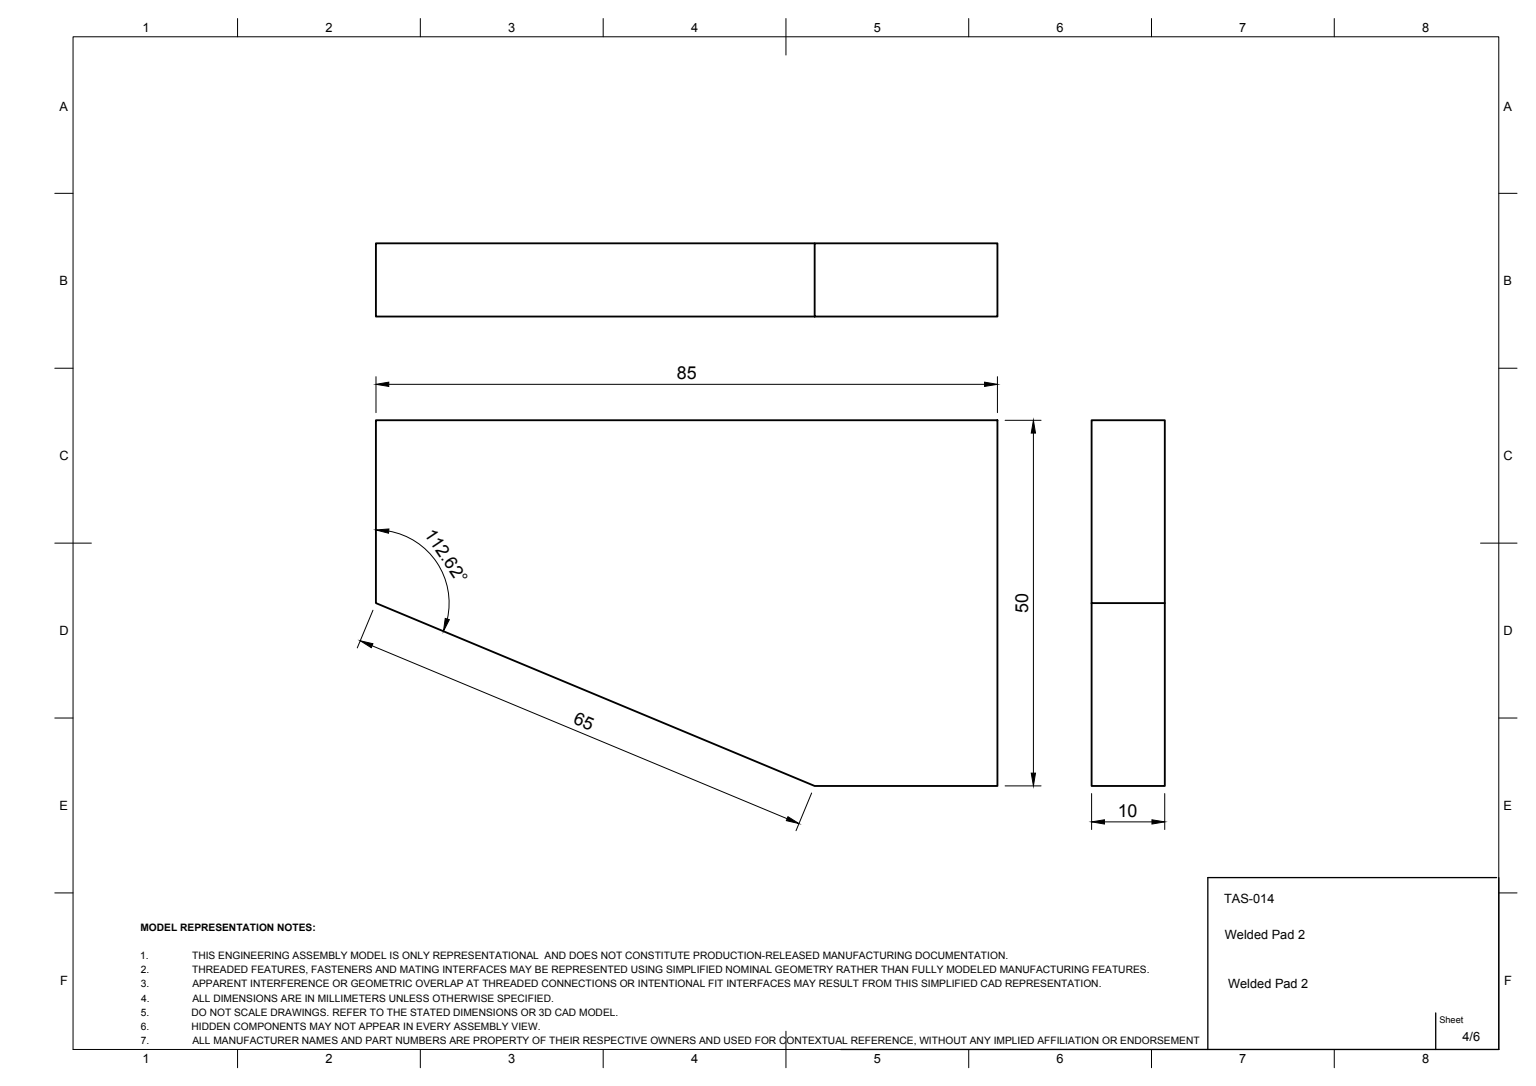
ISO-10303-21;
HEADER;
/* Generated by software containing ST-Developer
 * from STEP Tools, Inc. (www.steptools.com) 
 */

FILE_DESCRIPTION(
/* description */ ('STEP AP214'),
/* implementation_level */ '2;1');

FILE_NAME(
/* name */ 'Welded Pad 2.step',
/* time_stamp */ '2026-11-15T15:22:30-08:00',
/* author */ (''),
/* organization */ (''),
/* preprocessor_version */ 'ST-DEVELOPER v20.2',
/* originating_system */ 'Autodesk Translation Framework v15.17.0.0',
/* authorisation */ '');

FILE_SCHEMA (('AUTOMOTIVE_DESIGN { 1 0 10303 214 3 1 1 }'));
ENDSEC;

DATA;
#10=MECHANICAL_DESIGN_GEOMETRIC_PRESENTATION_REPRESENTATION('',(#87),#3119);
#70=SHAPE_REPRESENTATION_RELATIONSHIP('SRR','None',#3152,#74);
#74=ADVANCED_BREP_SHAPE_REPRESENTATION('',(#94),#3118);
#87=STYLED_ITEM('',(#3178),#94);
#94=MANIFOLD_SOLID_BREP('Body1',#1806);
#293=FACE_OUTER_BOUND('',#394,.T.);
#294=FACE_OUTER_BOUND('',#395,.T.);
#295=FACE_OUTER_BOUND('',#396,.T.);
#296=FACE_OUTER_BOUND('',#397,.T.);
#297=FACE_OUTER_BOUND('',#398,.T.);
#298=FACE_OUTER_BOUND('',#399,.T.);
#299=FACE_OUTER_BOUND('',#400,.T.);
#394=EDGE_LOOP('',(#1616,#1617,#1618,#1619));
#395=EDGE_LOOP('',(#1620,#1621,#1622,#1623));
#396=EDGE_LOOP('',(#1624,#1625,#1626,#1627));
#397=EDGE_LOOP('',(#1628,#1629,#1630,#1631));
#398=EDGE_LOOP('',(#1632,#1633,#1634,#1635));
#399=EDGE_LOOP('',(#1636,#1637,#1638,#1639,#1640));
#400=EDGE_LOOP('',(#1641,#1642,#1643,#1644,#1645));
#561=LINE('',#3065,#736);
#562=LINE('',#3067,#737);
#563=LINE('',#3069,#738);
#564=LINE('',#3070,#739);
#565=LINE('',#3073,#740);
#566=LINE('',#3075,#741);
#567=LINE('',#3076,#742);
#568=LINE('',#3079,#743);
#569=LINE('',#3081,#744);
#570=LINE('',#3082,#745);
#571=LINE('',#3085,#746);
#572=LINE('',#3087,#747);
#573=LINE('',#3088,#748);
#574=LINE('',#3090,#749);
#575=LINE('',#3091,#750);
#736=VECTOR('',#2524,1000.);
#737=VECTOR('',#2525,1000.);
#738=VECTOR('',#2526,1000.);
#739=VECTOR('',#2527,1000.);
#740=VECTOR('',#2530,1000.);
#741=VECTOR('',#2531,1000.);
#742=VECTOR('',#2532,1000.);
#743=VECTOR('',#2535,1000.);
#744=VECTOR('',#2536,1000.);
#745=VECTOR('',#2537,1000.);
#746=VECTOR('',#2540,1000.);
#747=VECTOR('',#2541,1000.);
#748=VECTOR('',#2542,1000.);
#749=VECTOR('',#2545,1000.);
#750=VECTOR('',#2546,1000.);
#911=VERTEX_POINT('',#3063);
#912=VERTEX_POINT('',#3064);
#913=VERTEX_POINT('',#3066);
#914=VERTEX_POINT('',#3068);
#915=VERTEX_POINT('',#3072);
#916=VERTEX_POINT('',#3074);
#917=VERTEX_POINT('',#3078);
#918=VERTEX_POINT('',#3080);
#919=VERTEX_POINT('',#3084);
#920=VERTEX_POINT('',#3086);
#1153=EDGE_CURVE('',#911,#912,#561,.T.);
#1154=EDGE_CURVE('',#913,#912,#562,.T.);
#1155=EDGE_CURVE('',#914,#913,#563,.T.);
#1156=EDGE_CURVE('',#914,#911,#564,.T.);
#1157=EDGE_CURVE('',#912,#915,#565,.T.);
#1158=EDGE_CURVE('',#916,#915,#566,.T.);
#1159=EDGE_CURVE('',#913,#916,#567,.T.);
#1160=EDGE_CURVE('',#915,#917,#568,.T.);
#1161=EDGE_CURVE('',#918,#917,#569,.T.);
#1162=EDGE_CURVE('',#916,#918,#570,.T.);
#1163=EDGE_CURVE('',#917,#919,#571,.T.);
#1164=EDGE_CURVE('',#920,#919,#572,.T.);
#1165=EDGE_CURVE('',#918,#920,#573,.T.);
#1166=EDGE_CURVE('',#919,#911,#574,.T.);
#1167=EDGE_CURVE('',#920,#914,#575,.T.);
#1616=ORIENTED_EDGE('',*,*,#1153,.T.);
#1617=ORIENTED_EDGE('',*,*,#1154,.F.);
#1618=ORIENTED_EDGE('',*,*,#1155,.F.);
#1619=ORIENTED_EDGE('',*,*,#1156,.T.);
#1620=ORIENTED_EDGE('',*,*,#1157,.T.);
#1621=ORIENTED_EDGE('',*,*,#1158,.F.);
#1622=ORIENTED_EDGE('',*,*,#1159,.F.);
#1623=ORIENTED_EDGE('',*,*,#1154,.T.);
#1624=ORIENTED_EDGE('',*,*,#1160,.T.);
#1625=ORIENTED_EDGE('',*,*,#1161,.F.);
#1626=ORIENTED_EDGE('',*,*,#1162,.F.);
#1627=ORIENTED_EDGE('',*,*,#1158,.T.);
#1628=ORIENTED_EDGE('',*,*,#1163,.T.);
#1629=ORIENTED_EDGE('',*,*,#1164,.F.);
#1630=ORIENTED_EDGE('',*,*,#1165,.F.);
#1631=ORIENTED_EDGE('',*,*,#1161,.T.);
#1632=ORIENTED_EDGE('',*,*,#1166,.T.);
#1633=ORIENTED_EDGE('',*,*,#1156,.F.);
#1634=ORIENTED_EDGE('',*,*,#1167,.F.);
#1635=ORIENTED_EDGE('',*,*,#1164,.T.);
#1636=ORIENTED_EDGE('',*,*,#1155,.T.);
#1637=ORIENTED_EDGE('',*,*,#1159,.T.);
#1638=ORIENTED_EDGE('',*,*,#1162,.T.);
#1639=ORIENTED_EDGE('',*,*,#1165,.T.);
#1640=ORIENTED_EDGE('',*,*,#1167,.T.);
#1641=ORIENTED_EDGE('',*,*,#1153,.F.);
#1642=ORIENTED_EDGE('',*,*,#1166,.F.);
#1643=ORIENTED_EDGE('',*,*,#1163,.F.);
#1644=ORIENTED_EDGE('',*,*,#1160,.F.);
#1645=ORIENTED_EDGE('',*,*,#1157,.F.);
#1700=PLANE('',#2015);
#1701=PLANE('',#2016);
#1702=PLANE('',#2017);
#1703=PLANE('',#2018);
#1704=PLANE('',#2019);
#1705=PLANE('',#2020);
#1706=PLANE('',#2021);
#1793=ADVANCED_FACE('',(#293),#1700,.F.);
#1794=ADVANCED_FACE('',(#294),#1701,.F.);
#1795=ADVANCED_FACE('',(#295),#1702,.F.);
#1796=ADVANCED_FACE('',(#296),#1703,.F.);
#1797=ADVANCED_FACE('',(#297),#1704,.F.);
#1798=ADVANCED_FACE('',(#298),#1705,.F.);
#1799=ADVANCED_FACE('',(#299),#1706,.T.);
#1806=CLOSED_SHELL('',(#1793,#1794,#1795,#1796,#1797,#1798,#1799));
#2014=AXIS2_PLACEMENT_3D('',#3061,#2520,#2521);
#2015=AXIS2_PLACEMENT_3D('',#3062,#2522,#2523);
#2016=AXIS2_PLACEMENT_3D('',#3071,#2528,#2529);
#2017=AXIS2_PLACEMENT_3D('',#3077,#2533,#2534);
#2018=AXIS2_PLACEMENT_3D('',#3083,#2538,#2539);
#2019=AXIS2_PLACEMENT_3D('',#3089,#2543,#2544);
#2020=AXIS2_PLACEMENT_3D('',#3092,#2547,#2548);
#2021=AXIS2_PLACEMENT_3D('',#3093,#2549,#2550);
#2520=DIRECTION('axis',(0.,0.,1.));
#2521=DIRECTION('refdir',(1.,0.,0.));
#2522=DIRECTION('center_axis',(0.,1.,0.));
#2523=DIRECTION('ref_axis',(0.,0.,1.));
#2524=DIRECTION('',(1.,0.,0.));
#2525=DIRECTION('',(0.,0.,-1.));
#2526=DIRECTION('',(1.,0.,0.));
#2527=DIRECTION('',(0.,0.,-1.));
#2528=DIRECTION('center_axis',(-1.,2.77555756156289E-16,0.));
#2529=DIRECTION('ref_axis',(-2.77555756156289E-16,-1.,0.));
#2530=DIRECTION('',(2.77555756156289E-16,1.,0.));
#2531=DIRECTION('',(0.,0.,-1.));
#2532=DIRECTION('',(2.77555756156289E-16,1.,0.));
#2533=DIRECTION('center_axis',(-0.923076923076923,-0.384615384615385,0.));
#2534=DIRECTION('ref_axis',(0.384615384615385,-0.923076923076923,0.));
#2535=DIRECTION('',(-0.384615384615385,0.923076923076923,0.));
#2536=DIRECTION('',(0.,0.,-1.));
#2537=DIRECTION('',(-0.384615384615385,0.923076923076923,0.));
#2538=DIRECTION('center_axis',(0.,-1.,0.));
#2539=DIRECTION('ref_axis',(0.,0.,-1.));
#2540=DIRECTION('',(-1.,0.,0.));
#2541=DIRECTION('',(0.,0.,-1.));
#2542=DIRECTION('',(-1.,0.,0.));
#2543=DIRECTION('center_axis',(1.,0.,0.));
#2544=DIRECTION('ref_axis',(0.,0.,-1.));
#2545=DIRECTION('',(0.,-1.,0.));
#2546=DIRECTION('',(0.,-1.,0.));
#2547=DIRECTION('center_axis',(0.,0.,-1.));
#2548=DIRECTION('ref_axis',(-1.,0.,0.));
#2549=DIRECTION('center_axis',(0.,0.,-1.));
#2550=DIRECTION('ref_axis',(-1.,0.,0.));
#3061=CARTESIAN_POINT('',(0.,0.,0.));
#3062=CARTESIAN_POINT('Origin',(50.,0.,5.));
#3063=CARTESIAN_POINT('',(0.,0.,-5.));
#3064=CARTESIAN_POINT('',(50.,0.,-5.));
#3065=CARTESIAN_POINT('',(50.,0.,-5.));
#3066=CARTESIAN_POINT('',(50.,0.,5.));
#3067=CARTESIAN_POINT('',(50.,0.,5.));
#3068=CARTESIAN_POINT('',(0.,0.,5.));
#3069=CARTESIAN_POINT('',(50.,0.,5.));
#3070=CARTESIAN_POINT('',(0.,0.,5.));
#3071=CARTESIAN_POINT('Origin',(50.,25.,5.));
#3072=CARTESIAN_POINT('',(50.,25.,-5.));
#3073=CARTESIAN_POINT('',(50.,25.,-5.));
#3074=CARTESIAN_POINT('',(50.,25.,5.));
#3075=CARTESIAN_POINT('',(50.,25.,5.));
#3076=CARTESIAN_POINT('',(50.,25.,5.));
#3077=CARTESIAN_POINT('Origin',(25.,85.,5.));
#3078=CARTESIAN_POINT('',(25.,85.,-5.));
#3079=CARTESIAN_POINT('',(25.,85.,-5.));
#3080=CARTESIAN_POINT('',(25.,85.,5.));
#3081=CARTESIAN_POINT('',(25.,85.,5.));
#3082=CARTESIAN_POINT('',(25.,85.,5.));
#3083=CARTESIAN_POINT('Origin',(0.,85.,5.));
#3084=CARTESIAN_POINT('',(0.,85.,-5.));
#3085=CARTESIAN_POINT('',(0.,85.,-5.));
#3086=CARTESIAN_POINT('',(0.,85.,5.));
#3087=CARTESIAN_POINT('',(0.,85.,5.));
#3088=CARTESIAN_POINT('',(0.,85.,5.));
#3089=CARTESIAN_POINT('Origin',(0.,0.,5.));
#3090=CARTESIAN_POINT('',(0.,0.,-5.));
#3091=CARTESIAN_POINT('',(0.,0.,5.));
#3092=CARTESIAN_POINT('Origin',(0.,0.,5.));
#3093=CARTESIAN_POINT('Origin',(0.,0.,-5.));
#3112=UNCERTAINTY_MEASURE_WITH_UNIT(LENGTH_MEASURE(0.01),#3120,
'DISTANCE_ACCURACY_VALUE',
'Maximum model space distance between geometric entities at asserted c
onnectivities');
#3113=UNCERTAINTY_MEASURE_WITH_UNIT(LENGTH_MEASURE(0.01),#3120,
'DISTANCE_ACCURACY_VALUE',
'Maximum model space distance between geometric entities at asserted c
onnectivities');
#3118=(
GEOMETRIC_REPRESENTATION_CONTEXT(3)
GLOBAL_UNCERTAINTY_ASSIGNED_CONTEXT((#3112))
GLOBAL_UNIT_ASSIGNED_CONTEXT((#3120,#3122,#3123))
REPRESENTATION_CONTEXT('','3D')
);
#3119=(
GEOMETRIC_REPRESENTATION_CONTEXT(3)
GLOBAL_UNCERTAINTY_ASSIGNED_CONTEXT((#3113))
GLOBAL_UNIT_ASSIGNED_CONTEXT((#3120,#3122,#3123))
REPRESENTATION_CONTEXT('','3D')
);
#3120=(
LENGTH_UNIT()
NAMED_UNIT(*)
SI_UNIT(.MILLI.,.METRE.)
);
#3122=(
NAMED_UNIT(*)
PLANE_ANGLE_UNIT()
SI_UNIT($,.RADIAN.)
);
#3123=(
NAMED_UNIT(*)
SI_UNIT($,.STERADIAN.)
SOLID_ANGLE_UNIT()
);
#3128=SHAPE_DEFINITION_REPRESENTATION(#3133,#3152);
#3133=PRODUCT_DEFINITION_SHAPE('',$,#3158);
#3152=SHAPE_REPRESENTATION('',(#2014),#3118);
#3153=PRODUCT_DEFINITION_CONTEXT('part definition',#3170,'design');
#3158=PRODUCT_DEFINITION('Welded Pad 2','Welded Pad 2',#3163,#3153);
#3163=PRODUCT_DEFINITION_FORMATION('',$,#3176);
#3170=APPLICATION_CONTEXT(
'Core Data for Automotive Mechanical Design Process');
#3171=PRODUCT_CONTEXT('part definition',#3170,'mechanical');
#3176=PRODUCT('Welded Pad 2','Welded Pad 2',$,(#3171));
#3178=PRESENTATION_STYLE_ASSIGNMENT((#3180));
#3180=SURFACE_STYLE_USAGE(.BOTH.,#3182);
#3182=SURFACE_SIDE_STYLE('',(#3184));
#3184=SURFACE_STYLE_FILL_AREA(#3186);
#3186=FILL_AREA_STYLE('Opaque(202,209,238)',(#3188));
#3188=FILL_AREA_STYLE_COLOUR('Opaque(202,209,238)',#3190);
#3190=COLOUR_RGB('Opaque(202,209,238)',0.792156862745098,0.819607843137255,
0.933333333333333);
ENDSEC;
END-ISO-10303-21;
